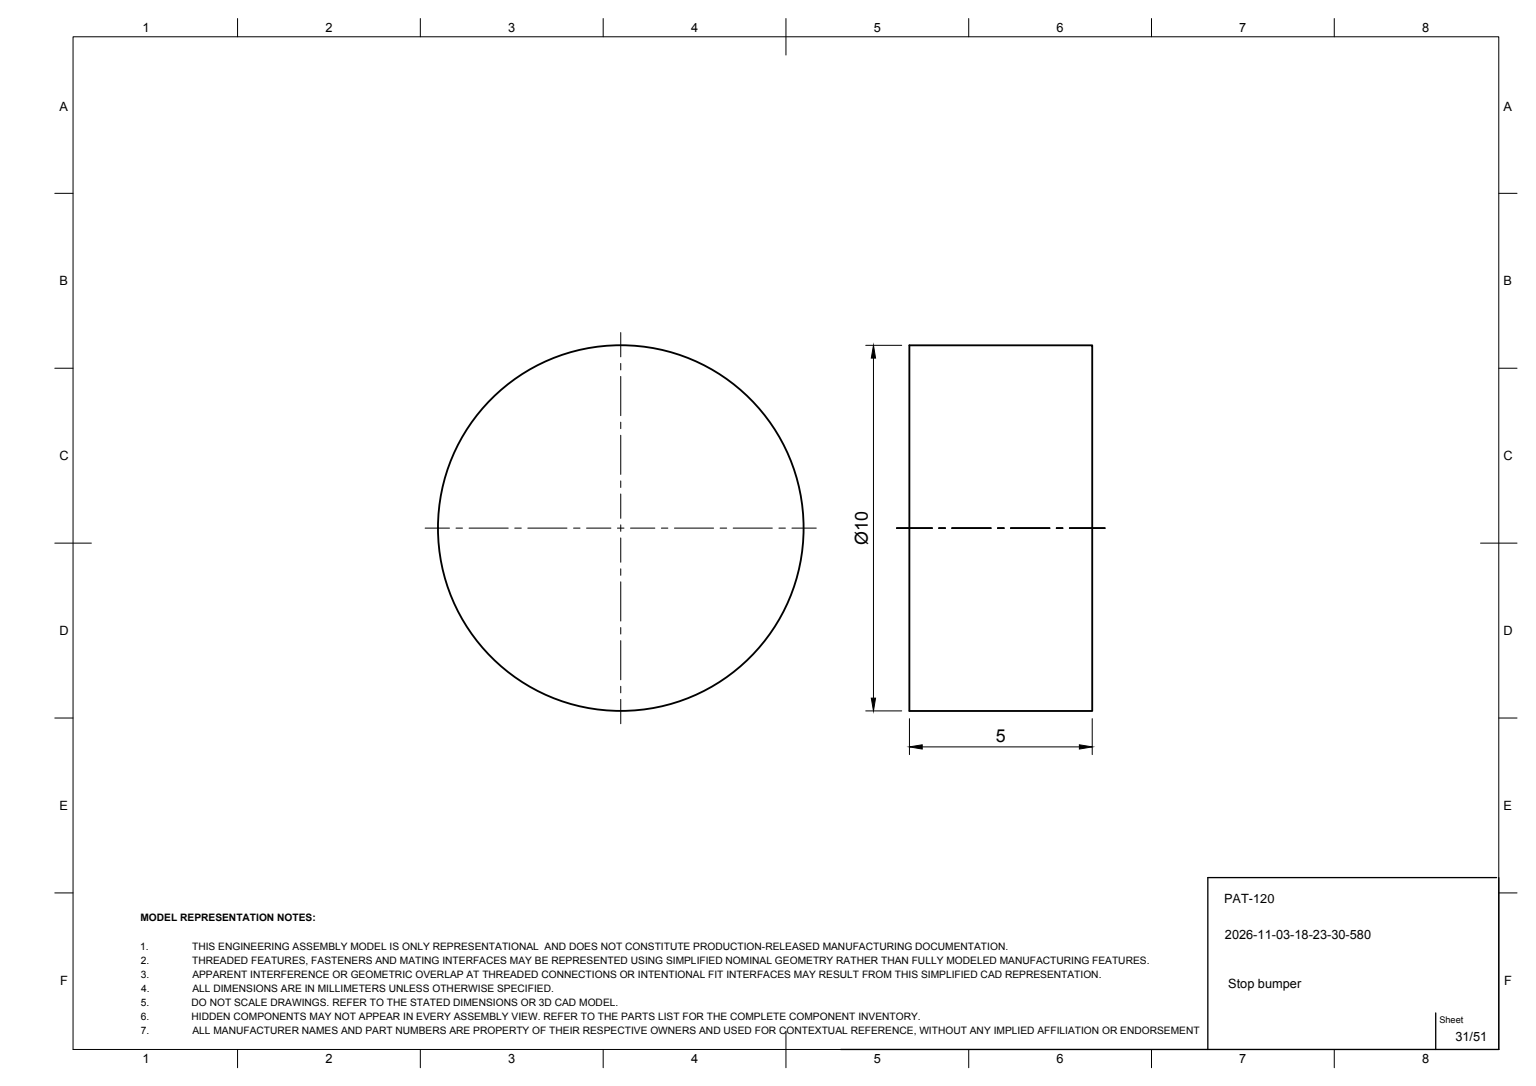
ISO-10303-21;
HEADER;
/* Generated by software containing ST-Developer
 * from STEP Tools, Inc. (www.steptools.com) 
 */

FILE_DESCRIPTION(
/* description */ ('Vibration shaker table dummy'),
/* implementation_level */ '2;1');

FILE_NAME(
/* name */ 'Stop bumper.step',
/* time_stamp */ '2026-10-27T10:55:14-07:00',
/* author */ (''),
/* organization */ (''),
/* preprocessor_version */ 'ST-DEVELOPER v20.2',
/* originating_system */ 'Autodesk Translation Framework v15.17.0.0',
/* authorisation */ '');

FILE_SCHEMA (('AUTOMOTIVE_DESIGN { 1 0 10303 214 3 1 1 }'));
ENDSEC;

DATA;
#10=MECHANICAL_DESIGN_GEOMETRIC_PRESENTATION_REPRESENTATION('',(#712),#22394);
#620=SHAPE_REPRESENTATION_RELATIONSHIP('SRR','None',#22666,#666);
#666=ADVANCED_BREP_SHAPE_REPRESENTATION('',(#758),#22372);
#712=STYLED_ITEM('',(#22975),#758);
#758=MANIFOLD_SOLID_BREP('Body1',#9230);
#1215=PLANE('',#10289);
#1216=PLANE('',#10290);
#1606=FACE_OUTER_BOUND('',#2273,.T.);
#1607=FACE_OUTER_BOUND('',#2274,.T.);
#1608=FACE_OUTER_BOUND('',#2275,.T.);
#2273=EDGE_LOOP('',(#7434,#7435,#7436,#7437));
#2274=EDGE_LOOP('',(#7438));
#2275=EDGE_LOOP('',(#7439));
#2976=LINE('',#21015,#3595);
#3595=VECTOR('',#12360,0.5);
#4096=CIRCLE('',#10287,0.5);
#4097=CIRCLE('',#10288,0.5);
#4763=VERTEX_POINT('',#21012);
#4764=VERTEX_POINT('',#21014);
#5710=EDGE_CURVE('',#4763,#4763,#4096,.T.);
#5711=EDGE_CURVE('',#4763,#4764,#2976,.T.);
#5712=EDGE_CURVE('',#4764,#4764,#4097,.T.);
#7434=ORIENTED_EDGE('',*,*,#5710,.F.);
#7435=ORIENTED_EDGE('',*,*,#5711,.T.);
#7436=ORIENTED_EDGE('',*,*,#5712,.T.);
#7437=ORIENTED_EDGE('',*,*,#5711,.F.);
#7438=ORIENTED_EDGE('',*,*,#5710,.T.);
#7439=ORIENTED_EDGE('',*,*,#5712,.F.);
#8612=CYLINDRICAL_SURFACE('',#10286,0.5);
#8971=ADVANCED_FACE('',(#1606),#8612,.T.);
#8972=ADVANCED_FACE('',(#1607),#1215,.T.);
#8973=ADVANCED_FACE('',(#1608),#1216,.F.);
#9230=CLOSED_SHELL('',(#8971,#8972,#8973));
#10285=AXIS2_PLACEMENT_3D('',#21010,#12354,#12355);
#10286=AXIS2_PLACEMENT_3D('',#21011,#12356,#12357);
#10287=AXIS2_PLACEMENT_3D('',#21013,#12358,#12359);
#10288=AXIS2_PLACEMENT_3D('',#21016,#12361,#12362);
#10289=AXIS2_PLACEMENT_3D('',#21017,#12363,#12364);
#10290=AXIS2_PLACEMENT_3D('',#21018,#12365,#12366);
#12354=DIRECTION('axis',(0.,0.,1.));
#12355=DIRECTION('refdir',(1.,0.,0.));
#12356=DIRECTION('center_axis',(0.,0.,1.));
#12357=DIRECTION('ref_axis',(1.,0.,0.));
#12358=DIRECTION('center_axis',(0.,0.,1.));
#12359=DIRECTION('ref_axis',(1.,0.,0.));
#12360=DIRECTION('',(0.,0.,-1.));
#12361=DIRECTION('center_axis',(0.,0.,1.));
#12362=DIRECTION('ref_axis',(1.,0.,0.));
#12363=DIRECTION('center_axis',(0.,0.,1.));
#12364=DIRECTION('ref_axis',(1.,0.,0.));
#12365=DIRECTION('center_axis',(0.,0.,1.));
#12366=DIRECTION('ref_axis',(1.,0.,0.));
#21010=CARTESIAN_POINT('',(0.,0.,0.));
#21011=CARTESIAN_POINT('Origin',(0.,-6.,13.6));
#21012=CARTESIAN_POINT('',(-0.5,-6.,14.1));
#21013=CARTESIAN_POINT('Origin',(0.,-6.,14.1));
#21014=CARTESIAN_POINT('',(-0.5,-6.,13.6));
#21015=CARTESIAN_POINT('',(-0.5,-6.,13.6));
#21016=CARTESIAN_POINT('Origin',(0.,-6.,13.6));
#21017=CARTESIAN_POINT('Origin',(0.,-6.,14.1));
#21018=CARTESIAN_POINT('Origin',(0.,-6.,13.6));
#22321=UNCERTAINTY_MEASURE_WITH_UNIT(LENGTH_MEASURE(0.001),#22395,
'DISTANCE_ACCURACY_VALUE',
'Maximum model space distance between geometric entities at asserted c
onnectivities');
#22343=UNCERTAINTY_MEASURE_WITH_UNIT(LENGTH_MEASURE(0.001),#22395,
'DISTANCE_ACCURACY_VALUE',
'Maximum model space distance between geometric entities at asserted c
onnectivities');
#22372=(
GEOMETRIC_REPRESENTATION_CONTEXT(3)
GLOBAL_UNCERTAINTY_ASSIGNED_CONTEXT((#22321))
GLOBAL_UNIT_ASSIGNED_CONTEXT((#22395,#22397,#22398))
REPRESENTATION_CONTEXT('','3D')
);
#22394=(
GEOMETRIC_REPRESENTATION_CONTEXT(3)
GLOBAL_UNCERTAINTY_ASSIGNED_CONTEXT((#22343))
GLOBAL_UNIT_ASSIGNED_CONTEXT((#22395,#22397,#22398))
REPRESENTATION_CONTEXT('','3D')
);
#22395=(
LENGTH_UNIT()
NAMED_UNIT(*)
SI_UNIT(.CENTI.,.METRE.)
);
#22397=(
NAMED_UNIT(*)
PLANE_ANGLE_UNIT()
SI_UNIT($,.RADIAN.)
);
#22398=(
NAMED_UNIT(*)
SI_UNIT($,.STERADIAN.)
SOLID_ANGLE_UNIT()
);
#22427=SHAPE_DEFINITION_REPRESENTATION(#22477,#22666);
#22477=PRODUCT_DEFINITION_SHAPE('',$,#22717);
#22666=SHAPE_REPRESENTATION('',(#10285),#22372);
#22688=PRODUCT_DEFINITION_CONTEXT('part definition',#22840,'design');
#22717=PRODUCT_DEFINITION('Stop bumper','Stop bumper',#22767,#22688);
#22767=PRODUCT_DEFINITION_FORMATION('',$,#22870);
#22840=APPLICATION_CONTEXT(
'Core Data for Automotive Mechanical Design Process');
#22841=PRODUCT_CONTEXT('part definition',#22840,'mechanical');
#22870=PRODUCT('Stop bumper','Stop bumper','Stop bumper',(#22841));
#22969=COLOUR_RGB('Off White',0.89,0.88,0.83);
#22970=FILL_AREA_STYLE_COLOUR('',#22969);
#22971=FILL_AREA_STYLE('',(#22970));
#22972=SURFACE_STYLE_FILL_AREA(#22971);
#22973=SURFACE_SIDE_STYLE('',(#22972));
#22974=SURFACE_STYLE_USAGE(.BOTH.,#22973);
#22975=PRESENTATION_STYLE_ASSIGNMENT((#22974));
ENDSEC;
END-ISO-10303-21;
